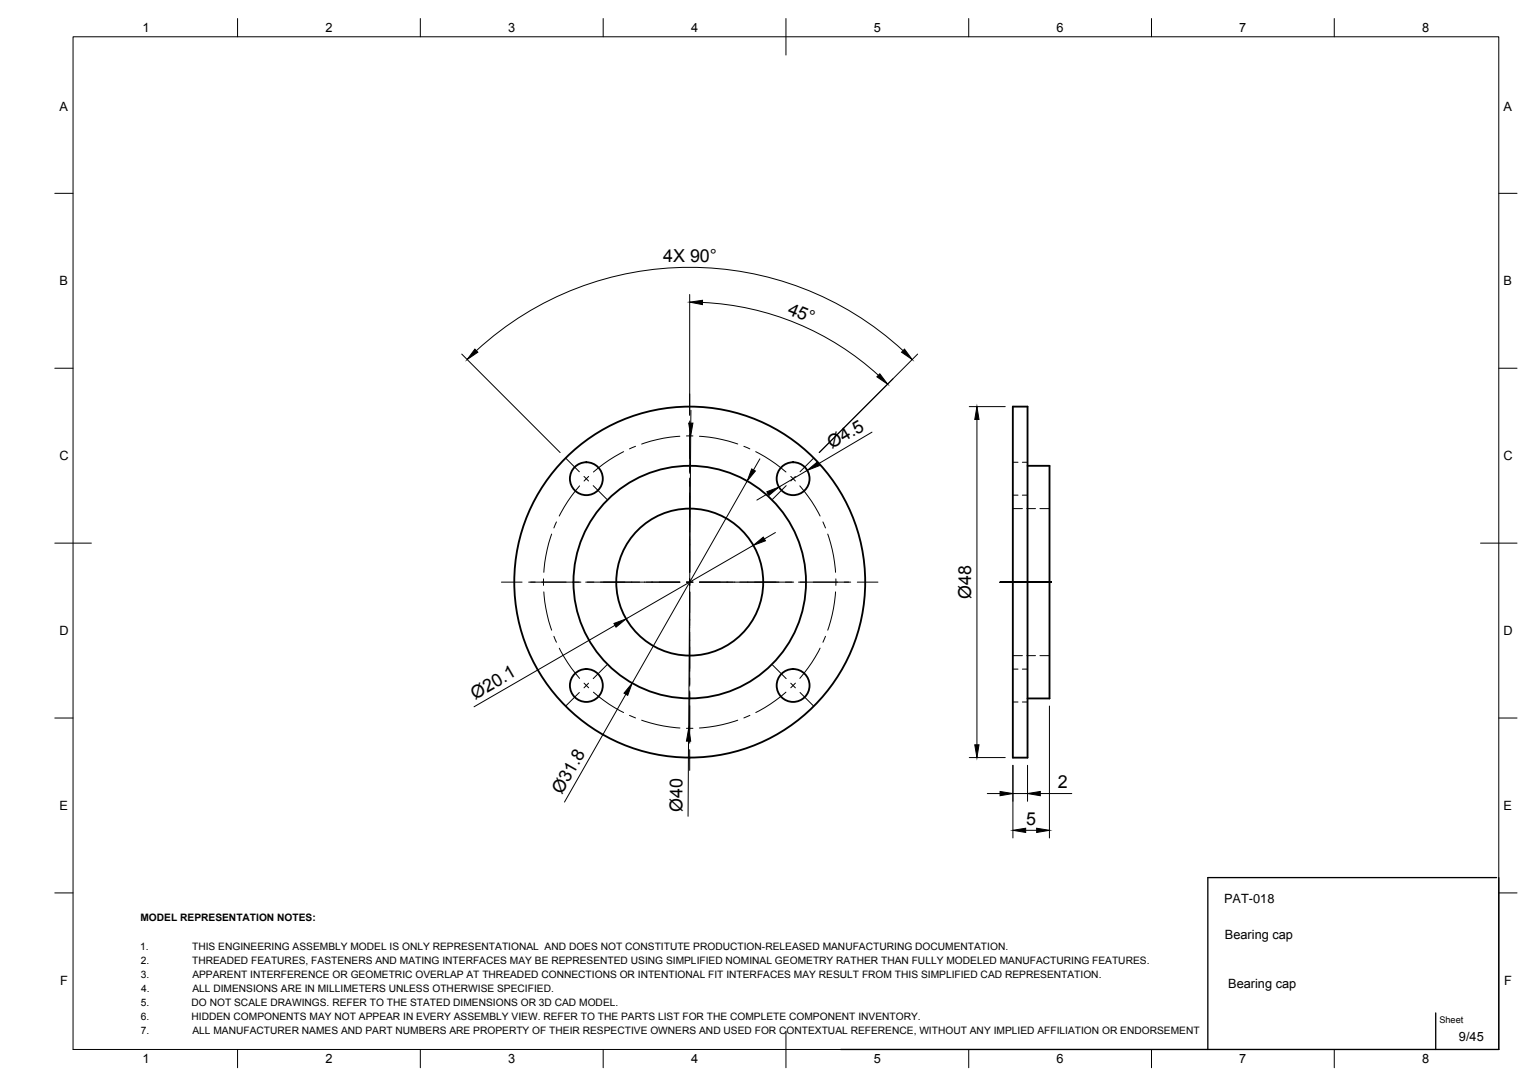
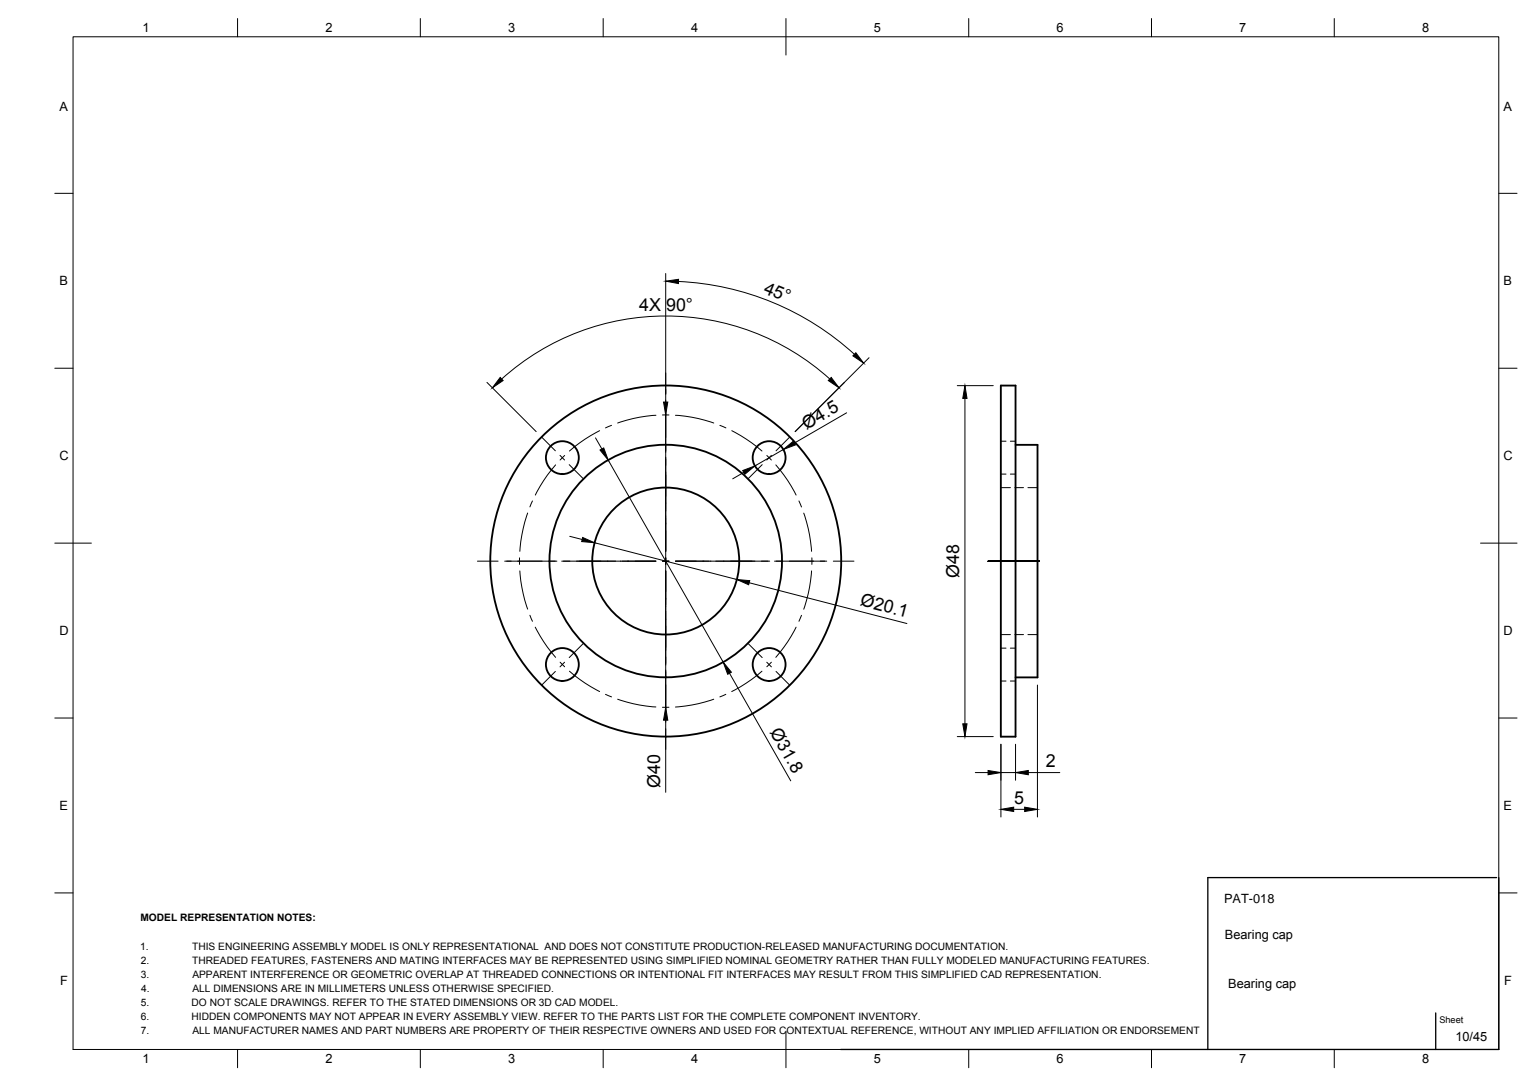
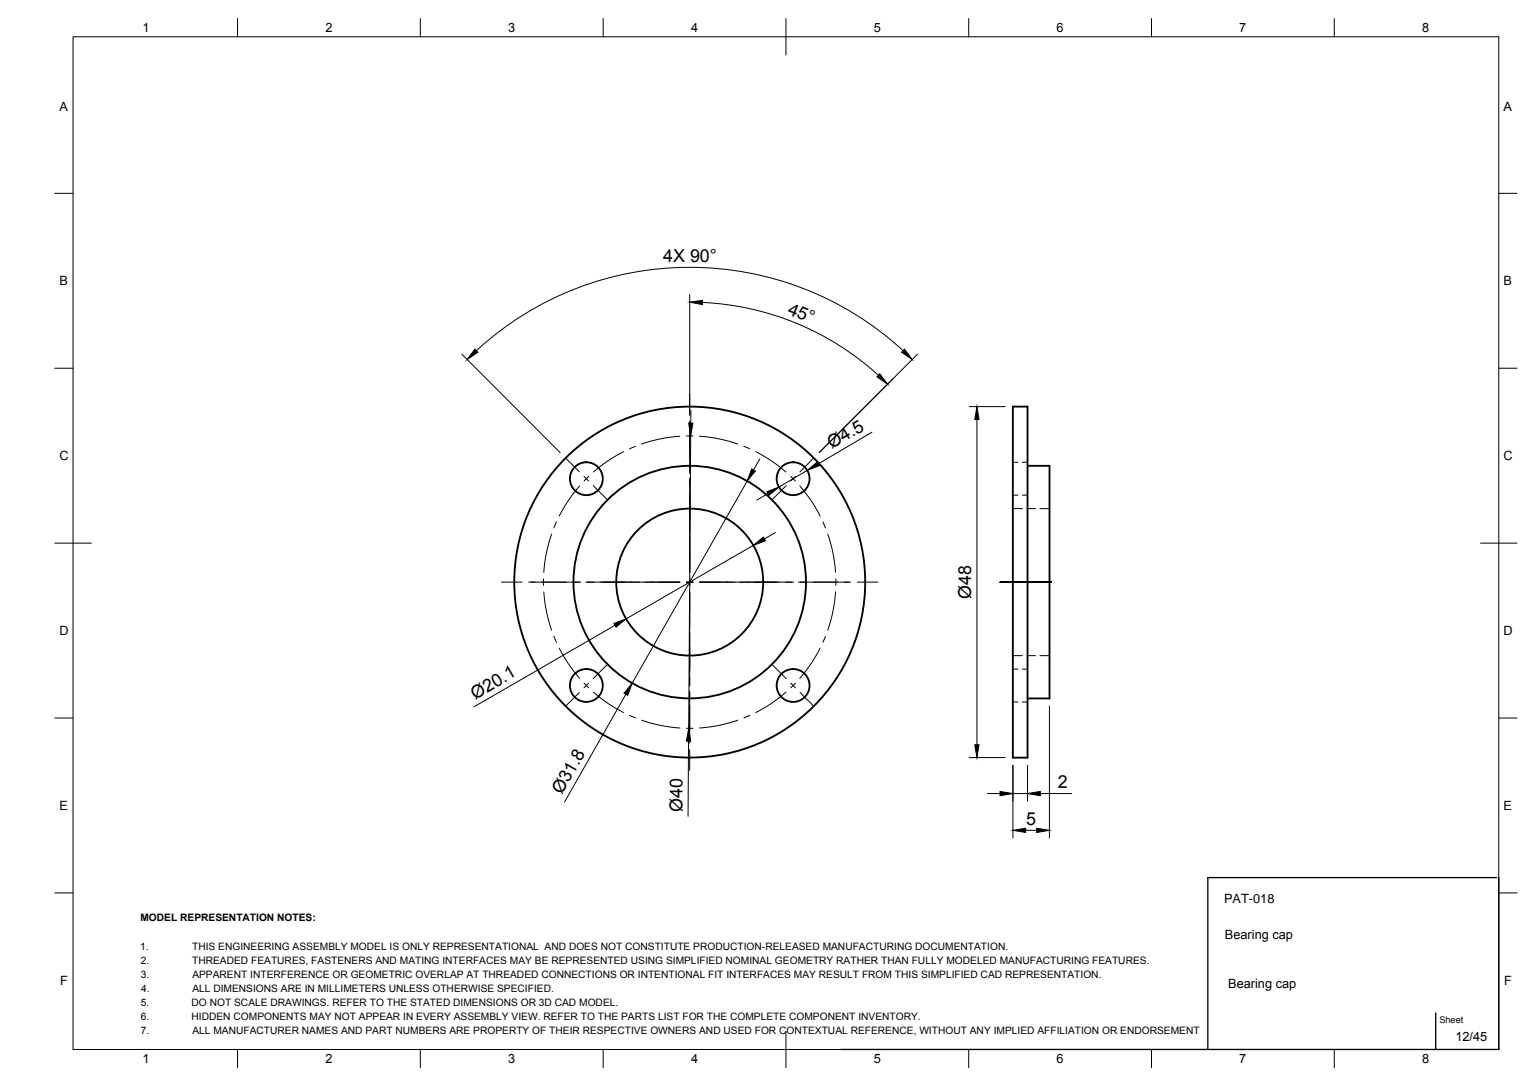
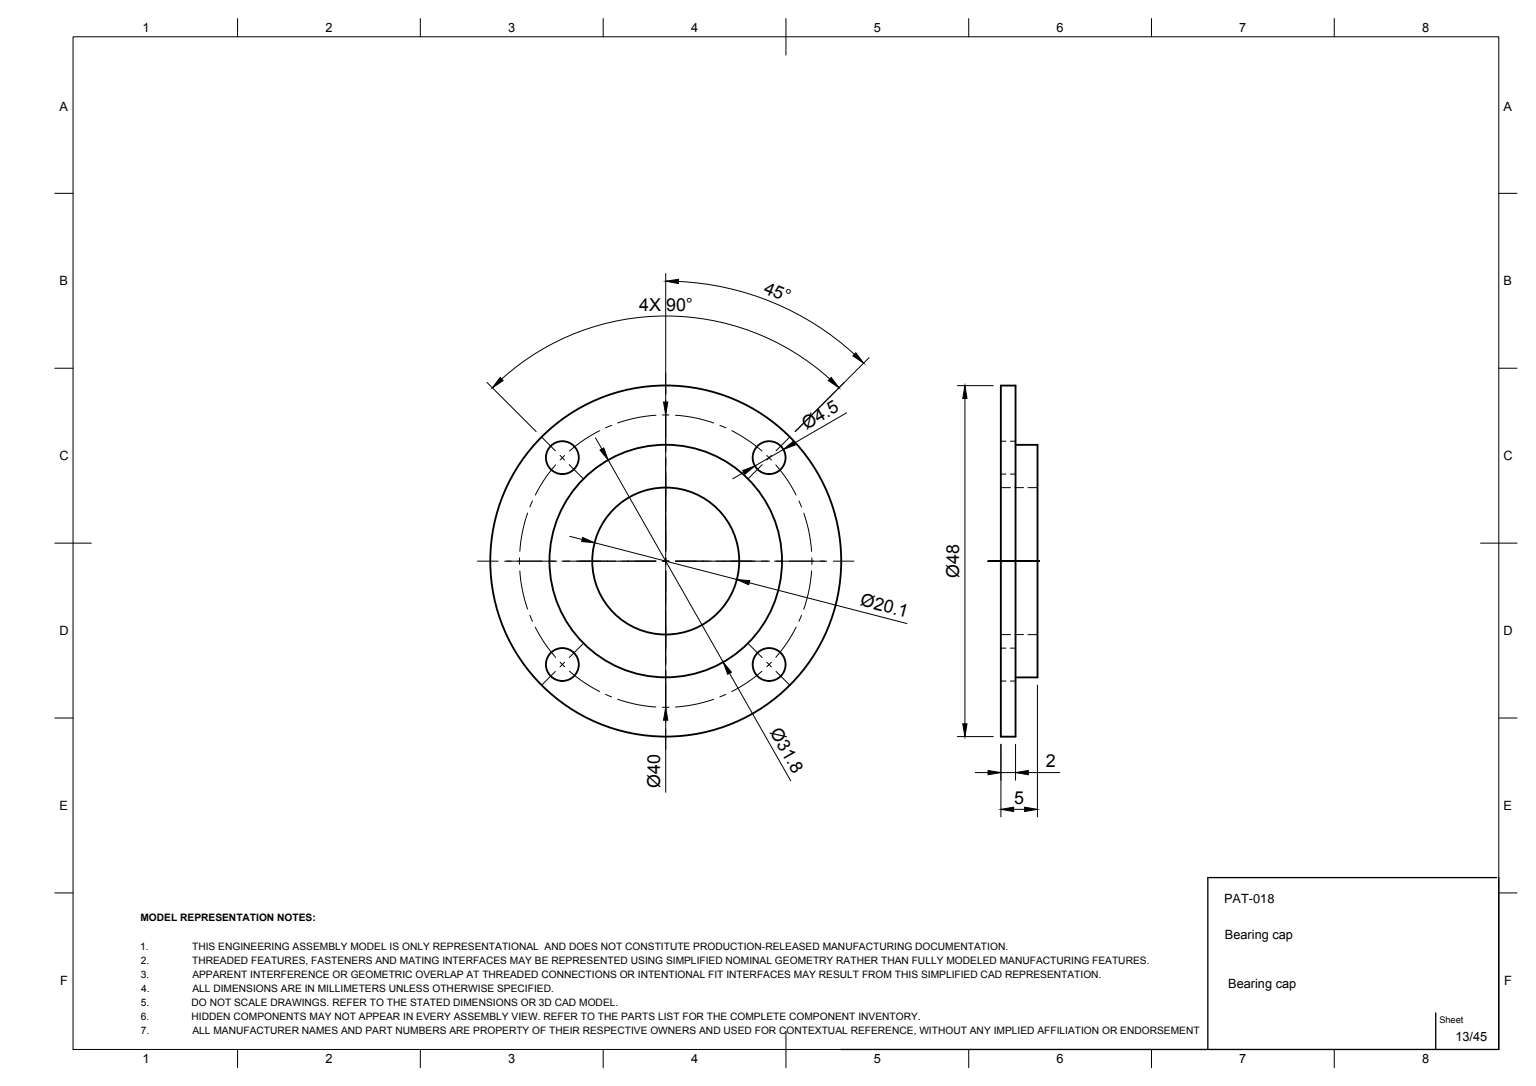
ISO-10303-21;
HEADER;
/* Generated by software containing ST-Developer
 * from STEP Tools, Inc. (www.steptools.com) 
 */

FILE_DESCRIPTION(
/* description */ ('Cam-driven reciprocating slide'),
/* implementation_level */ '2;1');

FILE_NAME(
/* name */ 'Bearing cap.step',
/* time_stamp */ '2026-10-28T03:25:20-07:00',
/* author */ (''),
/* organization */ (''),
/* preprocessor_version */ 'ST-DEVELOPER v20.2',
/* originating_system */ 'Autodesk Translation Framework v15.17.0.0',
/* authorisation */ '');

FILE_SCHEMA (('AUTOMOTIVE_DESIGN { 1 0 10303 214 3 1 1 }'));
ENDSEC;

DATA;
#10=MECHANICAL_DESIGN_GEOMETRIC_PRESENTATION_REPRESENTATION('',(#426),#13277);
#352=SHAPE_REPRESENTATION_RELATIONSHIP('SRR','None',#13445,#389);
#389=ADVANCED_BREP_SHAPE_REPRESENTATION('',(#470),#13240);
#426=STYLED_ITEM('',(#13720),#470);
#470=MANIFOLD_SOLID_BREP('Body1',#6402);
#534=FACE_BOUND('',#1359,.T.);
#535=FACE_BOUND('',#1363,.T.);
#536=FACE_BOUND('',#1364,.T.);
#537=FACE_BOUND('',#1365,.T.);
#538=FACE_BOUND('',#1366,.T.);
#539=FACE_BOUND('',#1367,.T.);
#540=FACE_BOUND('',#1369,.T.);
#541=FACE_BOUND('',#1370,.T.);
#542=FACE_BOUND('',#1371,.T.);
#543=FACE_BOUND('',#1372,.T.);
#544=FACE_BOUND('',#1373,.T.);
#714=PLANE('',#6947);
#715=PLANE('',#6954);
#716=PLANE('',#6955);
#947=FACE_OUTER_BOUND('',#1353,.T.);
#948=FACE_OUTER_BOUND('',#1354,.T.);
#949=FACE_OUTER_BOUND('',#1355,.T.);
#950=FACE_OUTER_BOUND('',#1356,.T.);
#951=FACE_OUTER_BOUND('',#1357,.T.);
#952=FACE_OUTER_BOUND('',#1358,.T.);
#953=FACE_OUTER_BOUND('',#1360,.T.);
#954=FACE_OUTER_BOUND('',#1361,.T.);
#955=FACE_OUTER_BOUND('',#1362,.T.);
#956=FACE_OUTER_BOUND('',#1368,.T.);
#1353=EDGE_LOOP('',(#4558,#4559,#4560,#4561));
#1354=EDGE_LOOP('',(#4562,#4563,#4564,#4565));
#1355=EDGE_LOOP('',(#4566,#4567,#4568,#4569));
#1356=EDGE_LOOP('',(#4570,#4571,#4572,#4573));
#1357=EDGE_LOOP('',(#4574,#4575,#4576,#4577));
#1358=EDGE_LOOP('',(#4578));
#1359=EDGE_LOOP('',(#4579));
#1360=EDGE_LOOP('',(#4580,#4581,#4582,#4583));
#1361=EDGE_LOOP('',(#4584,#4585,#4586,#4587));
#1362=EDGE_LOOP('',(#4588));
#1363=EDGE_LOOP('',(#4589));
#1364=EDGE_LOOP('',(#4590));
#1365=EDGE_LOOP('',(#4591));
#1366=EDGE_LOOP('',(#4592));
#1367=EDGE_LOOP('',(#4593));
#1368=EDGE_LOOP('',(#4594));
#1369=EDGE_LOOP('',(#4595));
#1370=EDGE_LOOP('',(#4596));
#1371=EDGE_LOOP('',(#4597));
#1372=EDGE_LOOP('',(#4598));
#1373=EDGE_LOOP('',(#4599));
#1918=LINE('',#9982,#2357);
#1919=LINE('',#9988,#2358);
#1920=LINE('',#9994,#2359);
#1921=LINE('',#10000,#2360);
#1922=LINE('',#10006,#2361);
#1923=LINE('',#10013,#2362);
#1924=LINE('',#10019,#2363);
#2357=VECTOR('',#7916,0.225);
#2358=VECTOR('',#7923,0.225);
#2359=VECTOR('',#7930,0.225);
#2360=VECTOR('',#7937,0.225);
#2361=VECTOR('',#7944,1.59);
#2362=VECTOR('',#7953,1.005);
#2363=VECTOR('',#7960,2.4);
#2737=CIRCLE('',#6933,0.225);
#2738=CIRCLE('',#6934,0.225);
#2739=CIRCLE('',#6936,0.225);
#2740=CIRCLE('',#6937,0.225);
#2741=CIRCLE('',#6939,0.225);
#2742=CIRCLE('',#6940,0.225);
#2743=CIRCLE('',#6942,0.225);
#2744=CIRCLE('',#6943,0.225);
#2745=CIRCLE('',#6945,1.59);
#2746=CIRCLE('',#6946,1.59);
#2747=CIRCLE('',#6948,1.005);
#2748=CIRCLE('',#6950,1.005);
#2749=CIRCLE('',#6952,2.4);
#2750=CIRCLE('',#6953,2.4);
#3109=VERTEX_POINT('',#9979);
#3110=VERTEX_POINT('',#9981);
#3111=VERTEX_POINT('',#9985);
#3112=VERTEX_POINT('',#9987);
#3113=VERTEX_POINT('',#9991);
#3114=VERTEX_POINT('',#9993);
#3115=VERTEX_POINT('',#9997);
#3116=VERTEX_POINT('',#9999);
#3117=VERTEX_POINT('',#10003);
#3118=VERTEX_POINT('',#10005);
#3119=VERTEX_POINT('',#10009);
#3120=VERTEX_POINT('',#10012);
#3121=VERTEX_POINT('',#10016);
#3122=VERTEX_POINT('',#10018);
#3669=EDGE_CURVE('',#3109,#3109,#2737,.T.);
#3670=EDGE_CURVE('',#3109,#3110,#1918,.T.);
#3671=EDGE_CURVE('',#3110,#3110,#2738,.T.);
#3672=EDGE_CURVE('',#3111,#3111,#2739,.T.);
#3673=EDGE_CURVE('',#3111,#3112,#1919,.T.);
#3674=EDGE_CURVE('',#3112,#3112,#2740,.T.);
#3675=EDGE_CURVE('',#3113,#3113,#2741,.T.);
#3676=EDGE_CURVE('',#3113,#3114,#1920,.T.);
#3677=EDGE_CURVE('',#3114,#3114,#2742,.T.);
#3678=EDGE_CURVE('',#3115,#3115,#2743,.T.);
#3679=EDGE_CURVE('',#3115,#3116,#1921,.T.);
#3680=EDGE_CURVE('',#3116,#3116,#2744,.T.);
#3681=EDGE_CURVE('',#3117,#3117,#2745,.T.);
#3682=EDGE_CURVE('',#3117,#3118,#1922,.T.);
#3683=EDGE_CURVE('',#3118,#3118,#2746,.T.);
#3684=EDGE_CURVE('',#3119,#3119,#2747,.T.);
#3685=EDGE_CURVE('',#3119,#3120,#1923,.T.);
#3686=EDGE_CURVE('',#3120,#3120,#2748,.T.);
#3687=EDGE_CURVE('',#3121,#3121,#2749,.T.);
#3688=EDGE_CURVE('',#3121,#3122,#1924,.T.);
#3689=EDGE_CURVE('',#3122,#3122,#2750,.T.);
#4558=ORIENTED_EDGE('',*,*,#3669,.F.);
#4559=ORIENTED_EDGE('',*,*,#3670,.T.);
#4560=ORIENTED_EDGE('',*,*,#3671,.F.);
#4561=ORIENTED_EDGE('',*,*,#3670,.F.);
#4562=ORIENTED_EDGE('',*,*,#3672,.F.);
#4563=ORIENTED_EDGE('',*,*,#3673,.T.);
#4564=ORIENTED_EDGE('',*,*,#3674,.F.);
#4565=ORIENTED_EDGE('',*,*,#3673,.F.);
#4566=ORIENTED_EDGE('',*,*,#3675,.F.);
#4567=ORIENTED_EDGE('',*,*,#3676,.T.);
#4568=ORIENTED_EDGE('',*,*,#3677,.F.);
#4569=ORIENTED_EDGE('',*,*,#3676,.F.);
#4570=ORIENTED_EDGE('',*,*,#3678,.F.);
#4571=ORIENTED_EDGE('',*,*,#3679,.T.);
#4572=ORIENTED_EDGE('',*,*,#3680,.F.);
#4573=ORIENTED_EDGE('',*,*,#3679,.F.);
#4574=ORIENTED_EDGE('',*,*,#3681,.F.);
#4575=ORIENTED_EDGE('',*,*,#3682,.T.);
#4576=ORIENTED_EDGE('',*,*,#3683,.F.);
#4577=ORIENTED_EDGE('',*,*,#3682,.F.);
#4578=ORIENTED_EDGE('',*,*,#3681,.T.);
#4579=ORIENTED_EDGE('',*,*,#3684,.T.);
#4580=ORIENTED_EDGE('',*,*,#3684,.F.);
#4581=ORIENTED_EDGE('',*,*,#3685,.T.);
#4582=ORIENTED_EDGE('',*,*,#3686,.T.);
#4583=ORIENTED_EDGE('',*,*,#3685,.F.);
#4584=ORIENTED_EDGE('',*,*,#3687,.F.);
#4585=ORIENTED_EDGE('',*,*,#3688,.T.);
#4586=ORIENTED_EDGE('',*,*,#3689,.T.);
#4587=ORIENTED_EDGE('',*,*,#3688,.F.);
#4588=ORIENTED_EDGE('',*,*,#3687,.T.);
#4589=ORIENTED_EDGE('',*,*,#3683,.T.);
#4590=ORIENTED_EDGE('',*,*,#3680,.T.);
#4591=ORIENTED_EDGE('',*,*,#3677,.T.);
#4592=ORIENTED_EDGE('',*,*,#3674,.T.);
#4593=ORIENTED_EDGE('',*,*,#3671,.T.);
#4594=ORIENTED_EDGE('',*,*,#3689,.F.);
#4595=ORIENTED_EDGE('',*,*,#3686,.F.);
#4596=ORIENTED_EDGE('',*,*,#3678,.T.);
#4597=ORIENTED_EDGE('',*,*,#3675,.T.);
#4598=ORIENTED_EDGE('',*,*,#3672,.T.);
#4599=ORIENTED_EDGE('',*,*,#3669,.T.);
#5905=CYLINDRICAL_SURFACE('',#6932,0.225);
#5906=CYLINDRICAL_SURFACE('',#6935,0.225);
#5907=CYLINDRICAL_SURFACE('',#6938,0.225);
#5908=CYLINDRICAL_SURFACE('',#6941,0.225);
#5909=CYLINDRICAL_SURFACE('',#6944,1.59);
#5910=CYLINDRICAL_SURFACE('',#6949,1.005);
#5911=CYLINDRICAL_SURFACE('',#6951,2.4);
#6065=ADVANCED_FACE('',(#947),#5905,.F.);
#6066=ADVANCED_FACE('',(#948),#5906,.F.);
#6067=ADVANCED_FACE('',(#949),#5907,.F.);
#6068=ADVANCED_FACE('',(#950),#5908,.F.);
#6069=ADVANCED_FACE('',(#951),#5909,.T.);
#6070=ADVANCED_FACE('',(#952,#534),#714,.T.);
#6071=ADVANCED_FACE('',(#953),#5910,.F.);
#6072=ADVANCED_FACE('',(#954),#5911,.T.);
#6073=ADVANCED_FACE('',(#955,#535,#536,#537,#538,#539),#715,.T.);
#6074=ADVANCED_FACE('',(#956,#540,#541,#542,#543,#544),#716,.F.);
#6402=CLOSED_SHELL('',(#6065,#6066,#6067,#6068,#6069,#6070,#6071,#6072,
#6073,#6074));
#6931=AXIS2_PLACEMENT_3D('',#9977,#7910,#7911);
#6932=AXIS2_PLACEMENT_3D('',#9978,#7912,#7913);
#6933=AXIS2_PLACEMENT_3D('',#9980,#7914,#7915);
#6934=AXIS2_PLACEMENT_3D('',#9983,#7917,#7918);
#6935=AXIS2_PLACEMENT_3D('',#9984,#7919,#7920);
#6936=AXIS2_PLACEMENT_3D('',#9986,#7921,#7922);
#6937=AXIS2_PLACEMENT_3D('',#9989,#7924,#7925);
#6938=AXIS2_PLACEMENT_3D('',#9990,#7926,#7927);
#6939=AXIS2_PLACEMENT_3D('',#9992,#7928,#7929);
#6940=AXIS2_PLACEMENT_3D('',#9995,#7931,#7932);
#6941=AXIS2_PLACEMENT_3D('',#9996,#7933,#7934);
#6942=AXIS2_PLACEMENT_3D('',#9998,#7935,#7936);
#6943=AXIS2_PLACEMENT_3D('',#10001,#7938,#7939);
#6944=AXIS2_PLACEMENT_3D('',#10002,#7940,#7941);
#6945=AXIS2_PLACEMENT_3D('',#10004,#7942,#7943);
#6946=AXIS2_PLACEMENT_3D('',#10007,#7945,#7946);
#6947=AXIS2_PLACEMENT_3D('',#10008,#7947,#7948);
#6948=AXIS2_PLACEMENT_3D('',#10010,#7949,#7950);
#6949=AXIS2_PLACEMENT_3D('',#10011,#7951,#7952);
#6950=AXIS2_PLACEMENT_3D('',#10014,#7954,#7955);
#6951=AXIS2_PLACEMENT_3D('',#10015,#7956,#7957);
#6952=AXIS2_PLACEMENT_3D('',#10017,#7958,#7959);
#6953=AXIS2_PLACEMENT_3D('',#10020,#7961,#7962);
#6954=AXIS2_PLACEMENT_3D('',#10021,#7963,#7964);
#6955=AXIS2_PLACEMENT_3D('',#10022,#7965,#7966);
#7910=DIRECTION('axis',(0.,0.,1.));
#7911=DIRECTION('refdir',(1.,0.,0.));
#7912=DIRECTION('center_axis',(0.,1.,0.));
#7913=DIRECTION('ref_axis',(1.,0.,0.));
#7914=DIRECTION('center_axis',(0.,1.,0.));
#7915=DIRECTION('ref_axis',(1.,0.,0.));
#7916=DIRECTION('',(0.,1.,0.));
#7917=DIRECTION('center_axis',(0.,-1.,0.));
#7918=DIRECTION('ref_axis',(1.,0.,0.));
#7919=DIRECTION('center_axis',(0.,1.,0.));
#7920=DIRECTION('ref_axis',(1.,0.,0.));
#7921=DIRECTION('center_axis',(0.,1.,0.));
#7922=DIRECTION('ref_axis',(1.,0.,0.));
#7923=DIRECTION('',(0.,1.,0.));
#7924=DIRECTION('center_axis',(0.,-1.,0.));
#7925=DIRECTION('ref_axis',(1.,0.,0.));
#7926=DIRECTION('center_axis',(0.,1.,0.));
#7927=DIRECTION('ref_axis',(1.,0.,0.));
#7928=DIRECTION('center_axis',(0.,1.,0.));
#7929=DIRECTION('ref_axis',(1.,0.,0.));
#7930=DIRECTION('',(0.,1.,0.));
#7931=DIRECTION('center_axis',(0.,-1.,0.));
#7932=DIRECTION('ref_axis',(1.,0.,0.));
#7933=DIRECTION('center_axis',(0.,1.,0.));
#7934=DIRECTION('ref_axis',(1.,0.,0.));
#7935=DIRECTION('center_axis',(0.,1.,0.));
#7936=DIRECTION('ref_axis',(1.,0.,0.));
#7937=DIRECTION('',(0.,1.,0.));
#7938=DIRECTION('center_axis',(0.,-1.,0.));
#7939=DIRECTION('ref_axis',(1.,0.,0.));
#7940=DIRECTION('center_axis',(0.,1.,0.));
#7941=DIRECTION('ref_axis',(1.,0.,0.));
#7942=DIRECTION('center_axis',(0.,1.,0.));
#7943=DIRECTION('ref_axis',(1.,0.,0.));
#7944=DIRECTION('',(0.,-1.,0.));
#7945=DIRECTION('center_axis',(0.,-1.,0.));
#7946=DIRECTION('ref_axis',(1.,0.,0.));
#7947=DIRECTION('center_axis',(0.,1.,0.));
#7948=DIRECTION('ref_axis',(1.,0.,0.));
#7949=DIRECTION('center_axis',(0.,-1.,0.));
#7950=DIRECTION('ref_axis',(1.,0.,0.));
#7951=DIRECTION('center_axis',(0.,1.,0.));
#7952=DIRECTION('ref_axis',(1.,0.,0.));
#7953=DIRECTION('',(0.,-1.,0.));
#7954=DIRECTION('center_axis',(0.,-1.,0.));
#7955=DIRECTION('ref_axis',(1.,0.,0.));
#7956=DIRECTION('center_axis',(0.,1.,0.));
#7957=DIRECTION('ref_axis',(1.,0.,0.));
#7958=DIRECTION('center_axis',(0.,1.,0.));
#7959=DIRECTION('ref_axis',(1.,0.,0.));
#7960=DIRECTION('',(0.,-1.,0.));
#7961=DIRECTION('center_axis',(0.,1.,0.));
#7962=DIRECTION('ref_axis',(1.,0.,0.));
#7963=DIRECTION('center_axis',(0.,1.,0.));
#7964=DIRECTION('ref_axis',(1.,0.,0.));
#7965=DIRECTION('center_axis',(0.,1.,0.));
#7966=DIRECTION('ref_axis',(1.,0.,0.));
#9977=CARTESIAN_POINT('',(0.,0.,0.));
#9978=CARTESIAN_POINT('Origin',(-1.4142135623731,-3.6,2.58578643762691));
#9979=CARTESIAN_POINT('',(-1.6392135623731,-3.5,2.58578643762691));
#9980=CARTESIAN_POINT('Origin',(-1.4142135623731,-3.5,2.58578643762691));
#9981=CARTESIAN_POINT('',(-1.6392135623731,-3.3,2.58578643762691));
#9982=CARTESIAN_POINT('',(-1.6392135623731,-3.6,2.58578643762691));
#9983=CARTESIAN_POINT('Origin',(-1.4142135623731,-3.3,2.58578643762691));
#9984=CARTESIAN_POINT('Origin',(-1.41421356237309,-3.6,5.41421356237309));
#9985=CARTESIAN_POINT('',(-1.6392135623731,-3.5,5.41421356237309));
#9986=CARTESIAN_POINT('Origin',(-1.41421356237309,-3.5,5.41421356237309));
#9987=CARTESIAN_POINT('',(-1.6392135623731,-3.3,5.41421356237309));
#9988=CARTESIAN_POINT('',(-1.6392135623731,-3.6,5.41421356237309));
#9989=CARTESIAN_POINT('Origin',(-1.41421356237309,-3.3,5.41421356237309));
#9990=CARTESIAN_POINT('Origin',(1.4142135623731,-3.6,5.41421356237309));
#9991=CARTESIAN_POINT('',(1.1892135623731,-3.5,5.41421356237309));
#9992=CARTESIAN_POINT('Origin',(1.4142135623731,-3.5,5.41421356237309));
#9993=CARTESIAN_POINT('',(1.1892135623731,-3.3,5.41421356237309));
#9994=CARTESIAN_POINT('',(1.1892135623731,-3.6,5.41421356237309));
#9995=CARTESIAN_POINT('Origin',(1.4142135623731,-3.3,5.41421356237309));
#9996=CARTESIAN_POINT('Origin',(1.41421356237309,-3.6,2.5857864376269));
#9997=CARTESIAN_POINT('',(1.18921356237309,-3.5,2.5857864376269));
#9998=CARTESIAN_POINT('Origin',(1.41421356237309,-3.5,2.5857864376269));
#9999=CARTESIAN_POINT('',(1.18921356237309,-3.3,2.5857864376269));
#10000=CARTESIAN_POINT('',(1.18921356237309,-3.6,2.5857864376269));
#10001=CARTESIAN_POINT('Origin',(1.41421356237309,-3.3,2.5857864376269));
#10002=CARTESIAN_POINT('Origin',(0.,-3.3,4.));
#10003=CARTESIAN_POINT('',(-1.59,-3.,4.));
#10004=CARTESIAN_POINT('Origin',(0.,-3.,4.));
#10005=CARTESIAN_POINT('',(-1.59,-3.3,4.));
#10006=CARTESIAN_POINT('',(-1.59,-3.3,4.));
#10007=CARTESIAN_POINT('Origin',(0.,-3.3,4.));
#10008=CARTESIAN_POINT('Origin',(0.,-3.,4.));
#10009=CARTESIAN_POINT('',(-1.005,-3.,4.));
#10010=CARTESIAN_POINT('Origin',(0.,-3.,4.));
#10011=CARTESIAN_POINT('Origin',(0.,-3.5,4.));
#10012=CARTESIAN_POINT('',(-1.005,-3.5,4.));
#10013=CARTESIAN_POINT('',(-1.005,-3.5,4.));
#10014=CARTESIAN_POINT('Origin',(0.,-3.5,4.));
#10015=CARTESIAN_POINT('Origin',(0.,-3.5,4.));
#10016=CARTESIAN_POINT('',(-2.4,-3.3,4.));
#10017=CARTESIAN_POINT('Origin',(0.,-3.3,4.));
#10018=CARTESIAN_POINT('',(-2.4,-3.5,4.));
#10019=CARTESIAN_POINT('',(-2.4,-3.5,4.));
#10020=CARTESIAN_POINT('Origin',(0.,-3.5,4.));
#10021=CARTESIAN_POINT('Origin',(0.,-3.3,4.));
#10022=CARTESIAN_POINT('Origin',(0.,-3.5,4.));
#13196=UNCERTAINTY_MEASURE_WITH_UNIT(LENGTH_MEASURE(0.001),#13278,
'DISTANCE_ACCURACY_VALUE',
'Maximum model space distance between geometric entities at asserted c
onnectivities');
#13233=UNCERTAINTY_MEASURE_WITH_UNIT(LENGTH_MEASURE(0.001),#13278,
'DISTANCE_ACCURACY_VALUE',
'Maximum model space distance between geometric entities at asserted c
onnectivities');
#13240=(
GEOMETRIC_REPRESENTATION_CONTEXT(3)
GLOBAL_UNCERTAINTY_ASSIGNED_CONTEXT((#13196))
GLOBAL_UNIT_ASSIGNED_CONTEXT((#13278,#13280,#13281))
REPRESENTATION_CONTEXT('','3D')
);
#13277=(
GEOMETRIC_REPRESENTATION_CONTEXT(3)
GLOBAL_UNCERTAINTY_ASSIGNED_CONTEXT((#13233))
GLOBAL_UNIT_ASSIGNED_CONTEXT((#13278,#13280,#13281))
REPRESENTATION_CONTEXT('','3D')
);
#13278=(
LENGTH_UNIT()
NAMED_UNIT(*)
SI_UNIT(.CENTI.,.METRE.)
);
#13280=(
NAMED_UNIT(*)
PLANE_ANGLE_UNIT()
SI_UNIT($,.RADIAN.)
);
#13281=(
NAMED_UNIT(*)
SI_UNIT($,.STERADIAN.)
SOLID_ANGLE_UNIT()
);
#13288=SHAPE_DEFINITION_REPRESENTATION(#13331,#13445);
#13331=PRODUCT_DEFINITION_SHAPE('',$,#13489);
#13445=SHAPE_REPRESENTATION('',(#6931),#13240);
#13482=PRODUCT_DEFINITION_CONTEXT('part definition',#13613,'design');
#13489=PRODUCT_DEFINITION('Bearing cap','Bearing cap',#13532,#13482);
#13532=PRODUCT_DEFINITION_FORMATION('',$,#13621);
#13613=APPLICATION_CONTEXT(
'Core Data for Automotive Mechanical Design Process');
#13614=PRODUCT_CONTEXT('part definition',#13613,'mechanical');
#13621=PRODUCT('Bearing cap','Bearing cap','Bearing cap',(#13614));
#13714=COLOUR_RGB('Grey',0.48,0.52,0.57);
#13715=FILL_AREA_STYLE_COLOUR('',#13714);
#13716=FILL_AREA_STYLE('',(#13715));
#13717=SURFACE_STYLE_FILL_AREA(#13716);
#13718=SURFACE_SIDE_STYLE('',(#13717));
#13719=SURFACE_STYLE_USAGE(.BOTH.,#13718);
#13720=PRESENTATION_STYLE_ASSIGNMENT((#13719));
ENDSEC;
END-ISO-10303-21;
